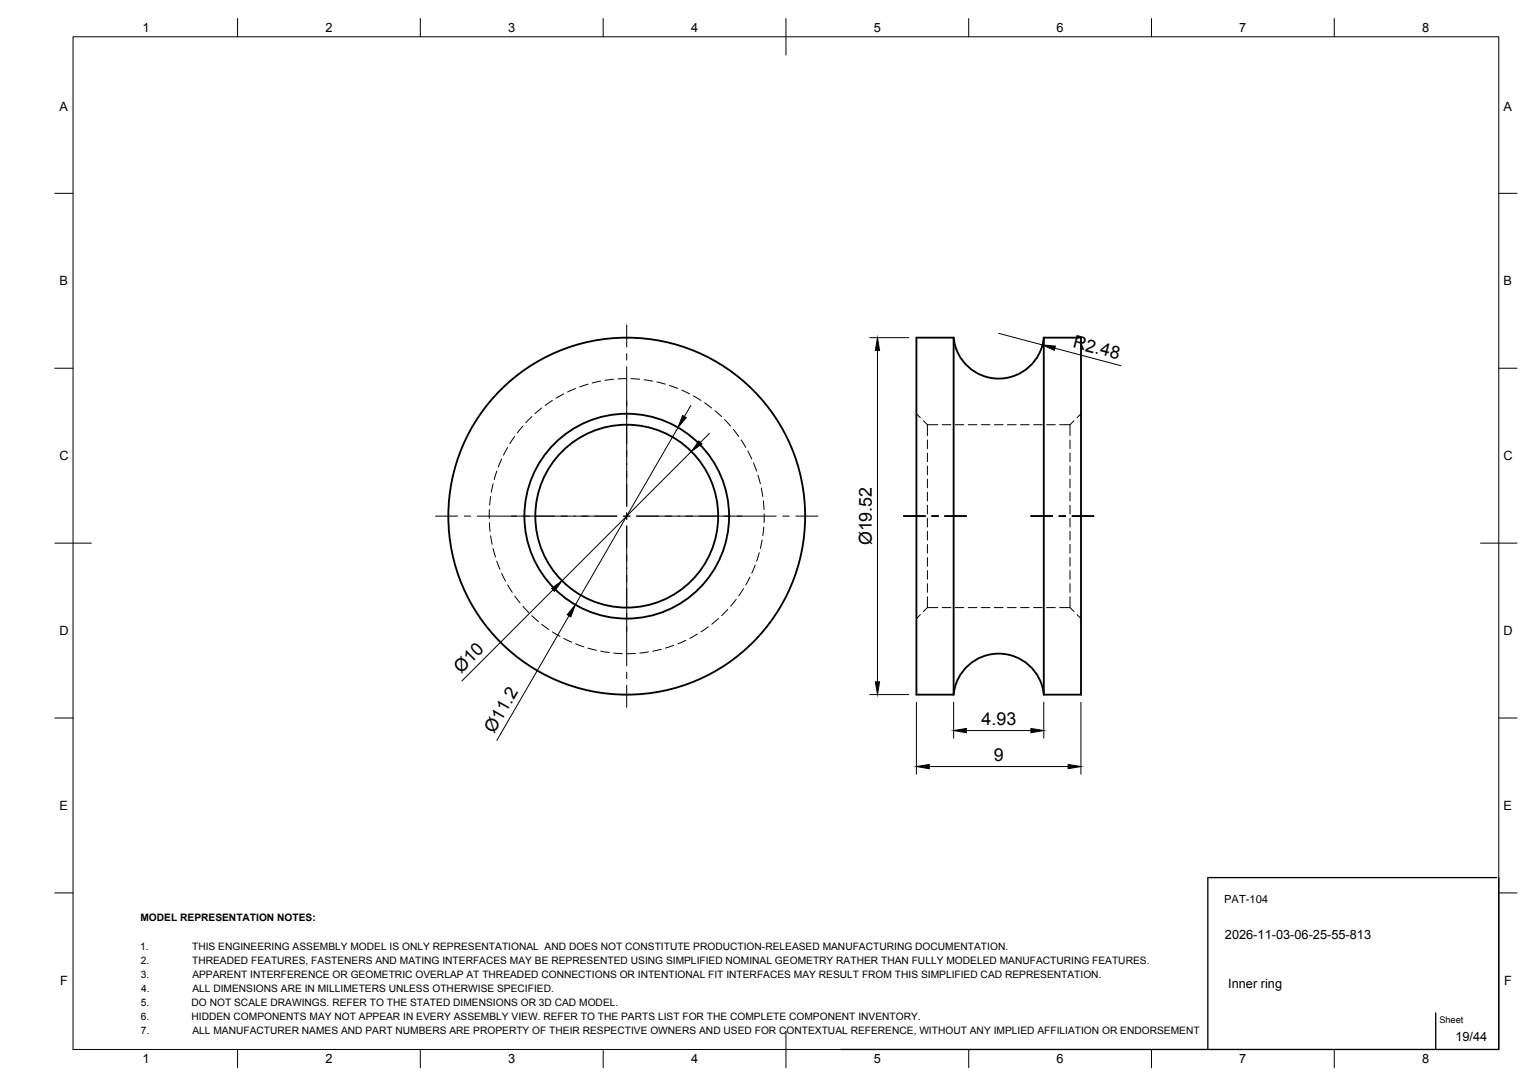
ISO-10303-21;
HEADER;
/* Generated by software containing ST-Developer
 * from STEP Tools, Inc. (www.steptools.com) 
 */

FILE_DESCRIPTION(
/* description */ ('Timing belt drive module 2 mm Pitch Timing 20T-40T'),

/* implementation_level */ '2;1');

FILE_NAME(
/* name */ 'Inner ring.step',
/* time_stamp */ '2026-10-28T03:25:12-07:00',
/* author */ (''),
/* organization */ (''),
/* preprocessor_version */ 'ST-DEVELOPER v20.2',
/* originating_system */ 'Autodesk Translation Framework v15.17.0.0',
/* authorisation */ '');

FILE_SCHEMA (('AUTOMOTIVE_DESIGN { 1 0 10303 214 3 1 1 }'));
ENDSEC;

DATA;
#10=MECHANICAL_DESIGN_GEOMETRIC_PRESENTATION_REPRESENTATION('',(#540),#17830);
#415=CONICAL_SURFACE('',#9889,0.53,0.785398163397448);
#416=CONICAL_SURFACE('',#9896,0.53,0.785398163397448);
#434=TOROIDAL_SURFACE('',#9878,1.,0.247676);
#454=SHAPE_REPRESENTATION_RELATIONSHIP('SRR','None',#18025,#497);
#497=ADVANCED_BREP_SHAPE_REPRESENTATION('',(#598),#17800);
#540=STYLED_ITEM('',(#18317),#598);
#598=MANIFOLD_SOLID_BREP('Body1',#8997);
#709=FACE_BOUND('',#1726,.T.);
#710=FACE_BOUND('',#1729,.T.);
#853=PLANE('',#9891);
#854=PLANE('',#9894);
#1128=FACE_OUTER_BOUND('',#1721,.T.);
#1129=FACE_OUTER_BOUND('',#1722,.T.);
#1130=FACE_OUTER_BOUND('',#1723,.T.);
#1131=FACE_OUTER_BOUND('',#1724,.T.);
#1132=FACE_OUTER_BOUND('',#1725,.T.);
#1133=FACE_OUTER_BOUND('',#1727,.T.);
#1134=FACE_OUTER_BOUND('',#1728,.T.);
#1135=FACE_OUTER_BOUND('',#1730,.T.);
#1721=EDGE_LOOP('',(#6541,#6542,#6543,#6544,#6545,#6546));
#1722=EDGE_LOOP('',(#6547,#6548,#6549,#6550,#6551));
#1723=EDGE_LOOP('',(#6552,#6553,#6554,#6555));
#1724=EDGE_LOOP('',(#6556,#6557,#6558,#6559));
#1725=EDGE_LOOP('',(#6560));
#1726=EDGE_LOOP('',(#6561));
#1727=EDGE_LOOP('',(#6562,#6563,#6564,#6565,#6566));
#1728=EDGE_LOOP('',(#6567));
#1729=EDGE_LOOP('',(#6568));
#1730=EDGE_LOOP('',(#6569,#6570,#6571,#6572));
#2316=CIRCLE('',#9879,0.976185);
#2317=CIRCLE('',#9880,0.976185);
#2318=CIRCLE('',#9881,0.247676);
#2319=CIRCLE('',#9882,0.976185);
#2320=CIRCLE('',#9883,0.976185);
#2321=CIRCLE('',#9885,0.976185);
#2322=CIRCLE('',#9887,0.5);
#2323=CIRCLE('',#9888,0.5);
#2324=CIRCLE('',#9890,0.56);
#2325=CIRCLE('',#9893,0.976185);
#2326=CIRCLE('',#9895,0.56);
#2998=LINE('',#14711,#3476);
#2999=LINE('',#14717,#3477);
#3000=LINE('',#14721,#3478);
#3001=LINE('',#14727,#3479);
#3002=LINE('',#14732,#3480);
#3476=VECTOR('',#11755,0.976185);
#3477=VECTOR('',#11762,0.5);
#3478=VECTOR('',#11767,0.53);
#3479=VECTOR('',#11776,0.976185);
#3480=VECTOR('',#11783,0.53);
#4002=VERTEX_POINT('',#14700);
#4003=VERTEX_POINT('',#14701);
#4004=VERTEX_POINT('',#14704);
#4005=VERTEX_POINT('',#14706);
#4006=VERTEX_POINT('',#14710);
#4007=VERTEX_POINT('',#14714);
#4008=VERTEX_POINT('',#14716);
#4009=VERTEX_POINT('',#14720);
#4010=VERTEX_POINT('',#14725);
#4011=VERTEX_POINT('',#14729);
#4953=EDGE_CURVE('',#4002,#4003,#2316,.T.);
#4954=EDGE_CURVE('',#4003,#4002,#2317,.T.);
#4955=EDGE_CURVE('',#4003,#4004,#2318,.T.);
#4956=EDGE_CURVE('',#4005,#4004,#2319,.T.);
#4957=EDGE_CURVE('',#4004,#4005,#2320,.T.);
#4958=EDGE_CURVE('',#4005,#4006,#2998,.T.);
#4959=EDGE_CURVE('',#4006,#4006,#2321,.T.);
#4960=EDGE_CURVE('',#4007,#4007,#2322,.T.);
#4961=EDGE_CURVE('',#4007,#4008,#2999,.T.);
#4962=EDGE_CURVE('',#4008,#4008,#2323,.T.);
#4963=EDGE_CURVE('',#4008,#4009,#3000,.T.);
#4964=EDGE_CURVE('',#4009,#4009,#2324,.T.);
#4965=EDGE_CURVE('',#4010,#4010,#2325,.T.);
#4966=EDGE_CURVE('',#4010,#4002,#3001,.T.);
#4967=EDGE_CURVE('',#4011,#4011,#2326,.T.);
#4968=EDGE_CURVE('',#4011,#4007,#3002,.T.);
#6541=ORIENTED_EDGE('',*,*,#4953,.F.);
#6542=ORIENTED_EDGE('',*,*,#4954,.F.);
#6543=ORIENTED_EDGE('',*,*,#4955,.T.);
#6544=ORIENTED_EDGE('',*,*,#4956,.F.);
#6545=ORIENTED_EDGE('',*,*,#4957,.F.);
#6546=ORIENTED_EDGE('',*,*,#4955,.F.);
#6547=ORIENTED_EDGE('',*,*,#4956,.T.);
#6548=ORIENTED_EDGE('',*,*,#4957,.T.);
#6549=ORIENTED_EDGE('',*,*,#4958,.T.);
#6550=ORIENTED_EDGE('',*,*,#4959,.T.);
#6551=ORIENTED_EDGE('',*,*,#4958,.F.);
#6552=ORIENTED_EDGE('',*,*,#4960,.T.);
#6553=ORIENTED_EDGE('',*,*,#4961,.T.);
#6554=ORIENTED_EDGE('',*,*,#4962,.F.);
#6555=ORIENTED_EDGE('',*,*,#4961,.F.);
#6556=ORIENTED_EDGE('',*,*,#4962,.T.);
#6557=ORIENTED_EDGE('',*,*,#4963,.T.);
#6558=ORIENTED_EDGE('',*,*,#4964,.F.);
#6559=ORIENTED_EDGE('',*,*,#4963,.F.);
#6560=ORIENTED_EDGE('',*,*,#4959,.F.);
#6561=ORIENTED_EDGE('',*,*,#4964,.T.);
#6562=ORIENTED_EDGE('',*,*,#4965,.F.);
#6563=ORIENTED_EDGE('',*,*,#4966,.T.);
#6564=ORIENTED_EDGE('',*,*,#4953,.T.);
#6565=ORIENTED_EDGE('',*,*,#4954,.T.);
#6566=ORIENTED_EDGE('',*,*,#4966,.F.);
#6567=ORIENTED_EDGE('',*,*,#4965,.T.);
#6568=ORIENTED_EDGE('',*,*,#4967,.F.);
#6569=ORIENTED_EDGE('',*,*,#4967,.T.);
#6570=ORIENTED_EDGE('',*,*,#4968,.T.);
#6571=ORIENTED_EDGE('',*,*,#4960,.F.);
#6572=ORIENTED_EDGE('',*,*,#4968,.F.);
#8267=CYLINDRICAL_SURFACE('',#9884,0.976185);
#8268=CYLINDRICAL_SURFACE('',#9886,0.5);
#8269=CYLINDRICAL_SURFACE('',#9892,0.976185);
#8626=ADVANCED_FACE('',(#1128),#434,.F.);
#8627=ADVANCED_FACE('',(#1129),#8267,.T.);
#8628=ADVANCED_FACE('',(#1130),#8268,.F.);
#8629=ADVANCED_FACE('',(#1131),#415,.F.);
#8630=ADVANCED_FACE('',(#1132,#709),#853,.T.);
#8631=ADVANCED_FACE('',(#1133),#8269,.T.);
#8632=ADVANCED_FACE('',(#1134,#710),#854,.T.);
#8633=ADVANCED_FACE('',(#1135),#416,.F.);
#8997=CLOSED_SHELL('',(#8626,#8627,#8628,#8629,#8630,#8631,#8632,#8633));
#9877=AXIS2_PLACEMENT_3D('',#14698,#11739,#11740);
#9878=AXIS2_PLACEMENT_3D('',#14699,#11741,#11742);
#9879=AXIS2_PLACEMENT_3D('',#14702,#11743,#11744);
#9880=AXIS2_PLACEMENT_3D('',#14703,#11745,#11746);
#9881=AXIS2_PLACEMENT_3D('',#14705,#11747,#11748);
#9882=AXIS2_PLACEMENT_3D('',#14707,#11749,#11750);
#9883=AXIS2_PLACEMENT_3D('',#14708,#11751,#11752);
#9884=AXIS2_PLACEMENT_3D('',#14709,#11753,#11754);
#9885=AXIS2_PLACEMENT_3D('',#14712,#11756,#11757);
#9886=AXIS2_PLACEMENT_3D('',#14713,#11758,#11759);
#9887=AXIS2_PLACEMENT_3D('',#14715,#11760,#11761);
#9888=AXIS2_PLACEMENT_3D('',#14718,#11763,#11764);
#9889=AXIS2_PLACEMENT_3D('',#14719,#11765,#11766);
#9890=AXIS2_PLACEMENT_3D('',#14722,#11768,#11769);
#9891=AXIS2_PLACEMENT_3D('',#14723,#11770,#11771);
#9892=AXIS2_PLACEMENT_3D('',#14724,#11772,#11773);
#9893=AXIS2_PLACEMENT_3D('',#14726,#11774,#11775);
#9894=AXIS2_PLACEMENT_3D('',#14728,#11777,#11778);
#9895=AXIS2_PLACEMENT_3D('',#14730,#11779,#11780);
#9896=AXIS2_PLACEMENT_3D('',#14731,#11781,#11782);
#11739=DIRECTION('axis',(0.,0.,1.));
#11740=DIRECTION('refdir',(1.,0.,0.));
#11741=DIRECTION('center_axis',(0.,-1.,0.));
#11742=DIRECTION('ref_axis',(0.,0.,-1.));
#11743=DIRECTION('center_axis',(0.,-1.,0.));
#11744=DIRECTION('ref_axis',(1.,0.,0.));
#11745=DIRECTION('center_axis',(0.,-1.,0.));
#11746=DIRECTION('ref_axis',(1.,0.,0.));
#11747=DIRECTION('center_axis',(1.,0.,1.22464679914735E-16));
#11748=DIRECTION('ref_axis',(-1.22464679914735E-16,0.,1.));
#11749=DIRECTION('center_axis',(0.,1.,0.));
#11750=DIRECTION('ref_axis',(1.,0.,0.));
#11751=DIRECTION('center_axis',(0.,1.,0.));
#11752=DIRECTION('ref_axis',(1.,0.,0.));
#11753=DIRECTION('center_axis',(0.,-1.,0.));
#11754=DIRECTION('ref_axis',(1.,0.,0.));
#11755=DIRECTION('',(0.,1.,0.));
#11756=DIRECTION('center_axis',(0.,-1.,0.));
#11757=DIRECTION('ref_axis',(1.,0.,0.));
#11758=DIRECTION('center_axis',(0.,-1.,0.));
#11759=DIRECTION('ref_axis',(1.,0.,0.));
#11760=DIRECTION('center_axis',(0.,-1.,0.));
#11761=DIRECTION('ref_axis',(1.,0.,0.));
#11762=DIRECTION('',(0.,1.,0.));
#11763=DIRECTION('center_axis',(0.,-1.,0.));
#11764=DIRECTION('ref_axis',(1.,0.,0.));
#11765=DIRECTION('center_axis',(0.,1.,0.));
#11766=DIRECTION('ref_axis',(1.,0.,0.));
#11767=DIRECTION('',(-0.707106781186547,0.707106781186548,-8.65956056235493E-17));
#11768=DIRECTION('center_axis',(0.,-1.,0.));
#11769=DIRECTION('ref_axis',(1.,0.,0.));
#11770=DIRECTION('center_axis',(0.,1.,0.));
#11771=DIRECTION('ref_axis',(0.,0.,1.));
#11772=DIRECTION('center_axis',(0.,-1.,0.));
#11773=DIRECTION('ref_axis',(1.,0.,0.));
#11774=DIRECTION('center_axis',(0.,-1.,0.));
#11775=DIRECTION('ref_axis',(1.,0.,0.));
#11776=DIRECTION('',(0.,1.,0.));
#11777=DIRECTION('center_axis',(0.,-1.,0.));
#11778=DIRECTION('ref_axis',(0.,0.,-1.));
#11779=DIRECTION('center_axis',(0.,-1.,0.));
#11780=DIRECTION('ref_axis',(1.,0.,0.));
#11781=DIRECTION('center_axis',(0.,-1.,0.));
#11782=DIRECTION('ref_axis',(1.,0.,0.));
#11783=DIRECTION('',(0.707106781186547,0.707106781186548,8.65956056235493E-17));
#14698=CARTESIAN_POINT('',(0.,0.,0.));
#14699=CARTESIAN_POINT('Origin',(0.,0.,0.));
#14700=CARTESIAN_POINT('',(-0.976185,-0.246528389340863,-1.19548183562566E-16));
#14701=CARTESIAN_POINT('',(-1.19548183562566E-16,-0.246528389340863,0.976185));
#14702=CARTESIAN_POINT('Origin',(0.,-0.246528389340863,0.));
#14703=CARTESIAN_POINT('Origin',(0.,-0.246528389340863,0.));
#14704=CARTESIAN_POINT('',(-1.19548183562566E-16,0.246528389340863,0.976185));
#14705=CARTESIAN_POINT('Origin',(-1.22464679914735E-16,0.,1.));
#14706=CARTESIAN_POINT('',(-0.976185,0.246528389340863,1.19548183562566E-16));
#14707=CARTESIAN_POINT('Origin',(0.,0.246528389340863,0.));
#14708=CARTESIAN_POINT('Origin',(0.,0.246528389340863,0.));
#14709=CARTESIAN_POINT('Origin',(0.,0.,0.));
#14710=CARTESIAN_POINT('',(-0.976185,0.45,-1.19548183562566E-16));
#14711=CARTESIAN_POINT('',(-0.976185,0.,-1.19548183562566E-16));
#14712=CARTESIAN_POINT('Origin',(0.,0.45,0.));
#14713=CARTESIAN_POINT('Origin',(0.,0.,0.));
#14714=CARTESIAN_POINT('',(-0.5,-0.39,-6.12323399573677E-17));
#14715=CARTESIAN_POINT('Origin',(0.,-0.39,0.));
#14716=CARTESIAN_POINT('',(-0.5,0.39,-6.12323399573677E-17));
#14717=CARTESIAN_POINT('',(-0.5,0.,-6.12323399573677E-17));
#14718=CARTESIAN_POINT('Origin',(0.,0.39,0.));
#14719=CARTESIAN_POINT('Origin',(0.,0.42,0.));
#14720=CARTESIAN_POINT('',(-0.56,0.45,-6.85802207522518E-17));
#14721=CARTESIAN_POINT('',(-0.53,0.42,-6.49062803548097E-17));
#14722=CARTESIAN_POINT('Origin',(0.,0.45,0.));
#14723=CARTESIAN_POINT('Origin',(0.976185,0.45,0.));
#14724=CARTESIAN_POINT('Origin',(0.,0.,0.));
#14725=CARTESIAN_POINT('',(-0.976185,-0.45,-1.19548183562566E-16));
#14726=CARTESIAN_POINT('Origin',(0.,-0.45,0.));
#14727=CARTESIAN_POINT('',(-0.976185,0.,-1.19548183562566E-16));
#14728=CARTESIAN_POINT('Origin',(0.56,-0.45,0.));
#14729=CARTESIAN_POINT('',(-0.56,-0.45,-6.85802207522518E-17));
#14730=CARTESIAN_POINT('Origin',(0.,-0.45,0.));
#14731=CARTESIAN_POINT('Origin',(0.,-0.42,0.));
#14732=CARTESIAN_POINT('',(-0.53,-0.42,-6.49062803548097E-17));
#17750=UNCERTAINTY_MEASURE_WITH_UNIT(LENGTH_MEASURE(0.001),#17831,
'DISTANCE_ACCURACY_VALUE',
'Maximum model space distance between geometric entities at asserted c
onnectivities');
#17780=UNCERTAINTY_MEASURE_WITH_UNIT(LENGTH_MEASURE(0.001),#17831,
'DISTANCE_ACCURACY_VALUE',
'Maximum model space distance between geometric entities at asserted c
onnectivities');
#17800=(
GEOMETRIC_REPRESENTATION_CONTEXT(3)
GLOBAL_UNCERTAINTY_ASSIGNED_CONTEXT((#17750))
GLOBAL_UNIT_ASSIGNED_CONTEXT((#17831,#17833,#17834))
REPRESENTATION_CONTEXT('','3D')
);
#17830=(
GEOMETRIC_REPRESENTATION_CONTEXT(3)
GLOBAL_UNCERTAINTY_ASSIGNED_CONTEXT((#17780))
GLOBAL_UNIT_ASSIGNED_CONTEXT((#17831,#17833,#17834))
REPRESENTATION_CONTEXT('','3D')
);
#17831=(
LENGTH_UNIT()
NAMED_UNIT(*)
SI_UNIT(.CENTI.,.METRE.)
);
#17833=(
NAMED_UNIT(*)
PLANE_ANGLE_UNIT()
SI_UNIT($,.RADIAN.)
);
#17834=(
NAMED_UNIT(*)
SI_UNIT($,.STERADIAN.)
SOLID_ANGLE_UNIT()
);
#17854=SHAPE_DEFINITION_REPRESENTATION(#17903,#18025);
#17903=PRODUCT_DEFINITION_SHAPE('',$,#18075);
#18025=SHAPE_REPRESENTATION('',(#9877),#17800);
#18055=PRODUCT_DEFINITION_CONTEXT('part definition',#18204,'design');
#18075=PRODUCT_DEFINITION('Inner ring','Inner ring',#18124,#18055);
#18124=PRODUCT_DEFINITION_FORMATION('',$,#18225);
#18204=APPLICATION_CONTEXT(
'Core Data for Automotive Mechanical Design Process');
#18205=PRODUCT_CONTEXT('part definition',#18204,'mechanical');
#18225=PRODUCT('Inner ring','Inner ring','Inner ring',(#18205));
#18311=COLOUR_RGB('Grey',0.48,0.52,0.57);
#18312=FILL_AREA_STYLE_COLOUR('',#18311);
#18313=FILL_AREA_STYLE('',(#18312));
#18314=SURFACE_STYLE_FILL_AREA(#18313);
#18315=SURFACE_SIDE_STYLE('',(#18314));
#18316=SURFACE_STYLE_USAGE(.BOTH.,#18315);
#18317=PRESENTATION_STYLE_ASSIGNMENT((#18316));
ENDSEC;
END-ISO-10303-21;
